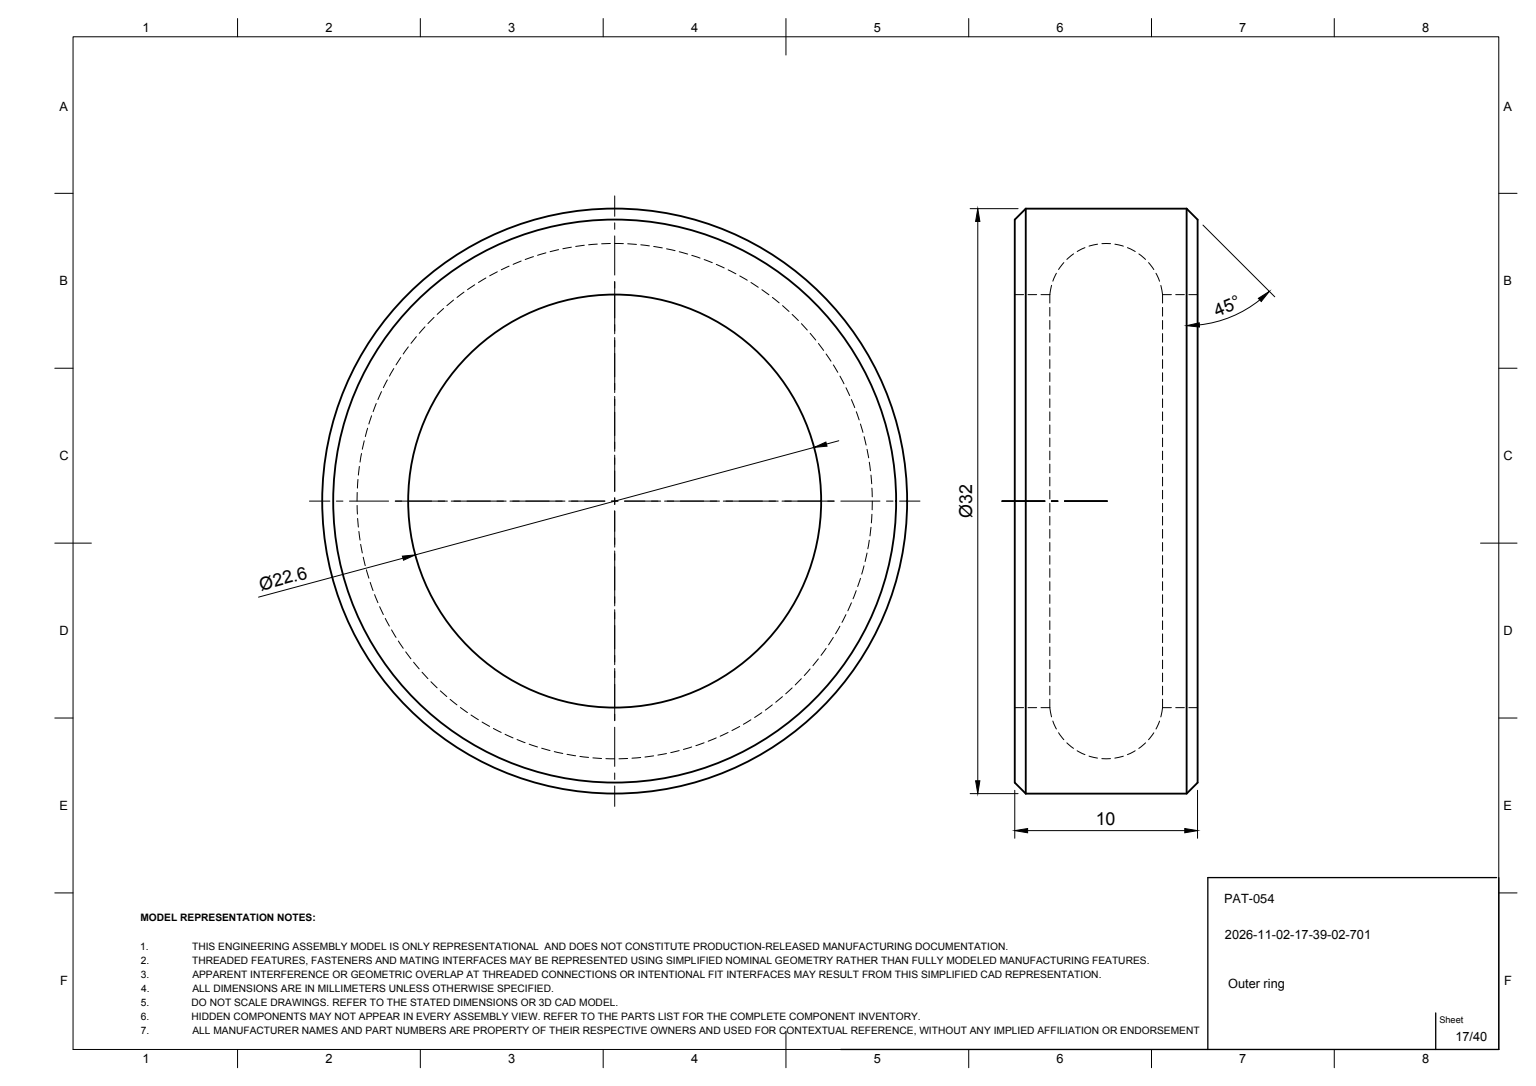
ISO-10303-21;
HEADER;
/* Generated by software containing ST-Developer
 * from STEP Tools, Inc. (www.steptools.com) 
 */

FILE_DESCRIPTION(
/* description */ ('PAT-054'),
/* implementation_level */ '2;1');

FILE_NAME(
/* name */ 'Outer ring.step',
/* time_stamp */ '2026-10-29T16:38:13-07:00',
/* author */ (''),
/* organization */ (''),
/* preprocessor_version */ 'ST-DEVELOPER v20.2',
/* originating_system */ 'Autodesk Translation Framework v15.17.0.0',
/* authorisation */ '');

FILE_SCHEMA (('AUTOMOTIVE_DESIGN { 1 0 10303 214 3 1 1 }'));
ENDSEC;

DATA;
#10=MECHANICAL_DESIGN_GEOMETRIC_PRESENTATION_REPRESENTATION('',(#909),#33981);
#779=CONICAL_SURFACE('',#13904,1.57,0.785398163397449);
#780=CONICAL_SURFACE('',#13908,1.57,0.785398163397449);
#808=TOROIDAL_SURFACE('',#13893,1.1,0.309556);
#821=SHAPE_REPRESENTATION_RELATIONSHIP('SRR','None',#34195,#865);
#865=ADVANCED_BREP_SHAPE_REPRESENTATION('',(#968),#33943);
#909=STYLED_ITEM('',(#34517),#968);
#968=MANIFOLD_SOLID_BREP('Body1',#13020);
#1130=FACE_BOUND('',#2580,.T.);
#1131=FACE_BOUND('',#2585,.T.);
#1313=PLANE('',#13901);
#1314=PLANE('',#13910);
#1736=FACE_OUTER_BOUND('',#2577,.T.);
#1737=FACE_OUTER_BOUND('',#2578,.T.);
#1738=FACE_OUTER_BOUND('',#2579,.T.);
#1739=FACE_OUTER_BOUND('',#2581,.T.);
#1740=FACE_OUTER_BOUND('',#2582,.T.);
#1741=FACE_OUTER_BOUND('',#2583,.T.);
#1742=FACE_OUTER_BOUND('',#2584,.T.);
#1743=FACE_OUTER_BOUND('',#2586,.T.);
#2577=EDGE_LOOP('',(#9259,#9260,#9261,#9262,#9263,#9264));
#2578=EDGE_LOOP('',(#9265,#9266,#9267,#9268,#9269));
#2579=EDGE_LOOP('',(#9270));
#2580=EDGE_LOOP('',(#9271));
#2581=EDGE_LOOP('',(#9272,#9273,#9274,#9275));
#2582=EDGE_LOOP('',(#9276,#9277,#9278,#9279));
#2583=EDGE_LOOP('',(#9280,#9281,#9282,#9283));
#2584=EDGE_LOOP('',(#9284));
#2585=EDGE_LOOP('',(#9285));
#2586=EDGE_LOOP('',(#9286,#9287,#9288,#9289,#9290));
#3463=LINE('',#19315,#4397);
#3464=LINE('',#19324,#4398);
#3465=LINE('',#19328,#4399);
#3466=LINE('',#19332,#4400);
#3467=LINE('',#19335,#4401);
#4397=VECTOR('',#15800,1.129765);
#4398=VECTOR('',#15811,1.57);
#4399=VECTOR('',#15816,1.6);
#4400=VECTOR('',#15821,1.57);
#4401=VECTOR('',#15826,1.129765);
#5264=CIRCLE('',#13894,1.129765);
#5265=CIRCLE('',#13895,1.129765);
#5266=CIRCLE('',#13896,0.309556);
#5267=CIRCLE('',#13897,1.129765);
#5268=CIRCLE('',#13898,1.129765);
#5269=CIRCLE('',#13900,1.129765);
#5270=CIRCLE('',#13902,1.54);
#5271=CIRCLE('',#13903,1.129765);
#5272=CIRCLE('',#13905,1.6);
#5273=CIRCLE('',#13907,1.6);
#5274=CIRCLE('',#13909,1.54);
#5826=VERTEX_POINT('',#19303);
#5827=VERTEX_POINT('',#19304);
#5828=VERTEX_POINT('',#19307);
#5829=VERTEX_POINT('',#19309);
#5830=VERTEX_POINT('',#19313);
#5831=VERTEX_POINT('',#19317);
#5832=VERTEX_POINT('',#19319);
#5833=VERTEX_POINT('',#19322);
#5834=VERTEX_POINT('',#19326);
#5835=VERTEX_POINT('',#19330);
#7129=EDGE_CURVE('',#5826,#5827,#5264,.T.);
#7130=EDGE_CURVE('',#5827,#5826,#5265,.T.);
#7131=EDGE_CURVE('',#5827,#5828,#5266,.T.);
#7132=EDGE_CURVE('',#5829,#5828,#5267,.T.);
#7133=EDGE_CURVE('',#5828,#5829,#5268,.T.);
#7134=EDGE_CURVE('',#5830,#5830,#5269,.T.);
#7135=EDGE_CURVE('',#5830,#5829,#3463,.T.);
#7136=EDGE_CURVE('',#5831,#5831,#5270,.T.);
#7137=EDGE_CURVE('',#5832,#5832,#5271,.T.);
#7138=EDGE_CURVE('',#5833,#5833,#5272,.T.);
#7139=EDGE_CURVE('',#5833,#5831,#3464,.T.);
#7140=EDGE_CURVE('',#5834,#5834,#5273,.T.);
#7141=EDGE_CURVE('',#5834,#5833,#3465,.T.);
#7142=EDGE_CURVE('',#5835,#5835,#5274,.T.);
#7143=EDGE_CURVE('',#5835,#5834,#3466,.T.);
#7144=EDGE_CURVE('',#5826,#5832,#3467,.T.);
#9259=ORIENTED_EDGE('',*,*,#7129,.F.);
#9260=ORIENTED_EDGE('',*,*,#7130,.F.);
#9261=ORIENTED_EDGE('',*,*,#7131,.T.);
#9262=ORIENTED_EDGE('',*,*,#7132,.F.);
#9263=ORIENTED_EDGE('',*,*,#7133,.F.);
#9264=ORIENTED_EDGE('',*,*,#7131,.F.);
#9265=ORIENTED_EDGE('',*,*,#7134,.T.);
#9266=ORIENTED_EDGE('',*,*,#7135,.T.);
#9267=ORIENTED_EDGE('',*,*,#7132,.T.);
#9268=ORIENTED_EDGE('',*,*,#7133,.T.);
#9269=ORIENTED_EDGE('',*,*,#7135,.F.);
#9270=ORIENTED_EDGE('',*,*,#7136,.F.);
#9271=ORIENTED_EDGE('',*,*,#7137,.T.);
#9272=ORIENTED_EDGE('',*,*,#7138,.F.);
#9273=ORIENTED_EDGE('',*,*,#7139,.T.);
#9274=ORIENTED_EDGE('',*,*,#7136,.T.);
#9275=ORIENTED_EDGE('',*,*,#7139,.F.);
#9276=ORIENTED_EDGE('',*,*,#7140,.F.);
#9277=ORIENTED_EDGE('',*,*,#7141,.T.);
#9278=ORIENTED_EDGE('',*,*,#7138,.T.);
#9279=ORIENTED_EDGE('',*,*,#7141,.F.);
#9280=ORIENTED_EDGE('',*,*,#7142,.F.);
#9281=ORIENTED_EDGE('',*,*,#7143,.T.);
#9282=ORIENTED_EDGE('',*,*,#7140,.T.);
#9283=ORIENTED_EDGE('',*,*,#7143,.F.);
#9284=ORIENTED_EDGE('',*,*,#7142,.T.);
#9285=ORIENTED_EDGE('',*,*,#7134,.F.);
#9286=ORIENTED_EDGE('',*,*,#7129,.T.);
#9287=ORIENTED_EDGE('',*,*,#7130,.T.);
#9288=ORIENTED_EDGE('',*,*,#7144,.T.);
#9289=ORIENTED_EDGE('',*,*,#7137,.F.);
#9290=ORIENTED_EDGE('',*,*,#7144,.F.);
#12052=CYLINDRICAL_SURFACE('',#13899,1.129765);
#12053=CYLINDRICAL_SURFACE('',#13906,1.6);
#12054=CYLINDRICAL_SURFACE('',#13911,1.129765);
#12448=ADVANCED_FACE('',(#1736),#808,.F.);
#12449=ADVANCED_FACE('',(#1737),#12052,.F.);
#12450=ADVANCED_FACE('',(#1738,#1130),#1313,.T.);
#12451=ADVANCED_FACE('',(#1739),#779,.T.);
#12452=ADVANCED_FACE('',(#1740),#12053,.T.);
#12453=ADVANCED_FACE('',(#1741),#780,.T.);
#12454=ADVANCED_FACE('',(#1742,#1131),#1314,.T.);
#12455=ADVANCED_FACE('',(#1743),#12054,.F.);
#13020=CLOSED_SHELL('',(#12448,#12449,#12450,#12451,#12452,#12453,#12454,
#12455));
#13892=AXIS2_PLACEMENT_3D('',#19301,#15782,#15783);
#13893=AXIS2_PLACEMENT_3D('',#19302,#15784,#15785);
#13894=AXIS2_PLACEMENT_3D('',#19305,#15786,#15787);
#13895=AXIS2_PLACEMENT_3D('',#19306,#15788,#15789);
#13896=AXIS2_PLACEMENT_3D('',#19308,#15790,#15791);
#13897=AXIS2_PLACEMENT_3D('',#19310,#15792,#15793);
#13898=AXIS2_PLACEMENT_3D('',#19311,#15794,#15795);
#13899=AXIS2_PLACEMENT_3D('',#19312,#15796,#15797);
#13900=AXIS2_PLACEMENT_3D('',#19314,#15798,#15799);
#13901=AXIS2_PLACEMENT_3D('',#19316,#15801,#15802);
#13902=AXIS2_PLACEMENT_3D('',#19318,#15803,#15804);
#13903=AXIS2_PLACEMENT_3D('',#19320,#15805,#15806);
#13904=AXIS2_PLACEMENT_3D('',#19321,#15807,#15808);
#13905=AXIS2_PLACEMENT_3D('',#19323,#15809,#15810);
#13906=AXIS2_PLACEMENT_3D('',#19325,#15812,#15813);
#13907=AXIS2_PLACEMENT_3D('',#19327,#15814,#15815);
#13908=AXIS2_PLACEMENT_3D('',#19329,#15817,#15818);
#13909=AXIS2_PLACEMENT_3D('',#19331,#15819,#15820);
#13910=AXIS2_PLACEMENT_3D('',#19333,#15822,#15823);
#13911=AXIS2_PLACEMENT_3D('',#19334,#15824,#15825);
#15782=DIRECTION('axis',(0.,0.,1.));
#15783=DIRECTION('refdir',(1.,0.,0.));
#15784=DIRECTION('center_axis',(0.,-1.,0.));
#15785=DIRECTION('ref_axis',(0.,0.,-1.));
#15786=DIRECTION('center_axis',(0.,-1.,0.));
#15787=DIRECTION('ref_axis',(1.,0.,0.));
#15788=DIRECTION('center_axis',(0.,-1.,0.));
#15789=DIRECTION('ref_axis',(1.,0.,0.));
#15790=DIRECTION('center_axis',(1.,0.,1.22464679914735E-16));
#15791=DIRECTION('ref_axis',(-1.22464679914735E-16,0.,1.));
#15792=DIRECTION('center_axis',(0.,1.,0.));
#15793=DIRECTION('ref_axis',(1.,0.,0.));
#15794=DIRECTION('center_axis',(0.,1.,0.));
#15795=DIRECTION('ref_axis',(1.,0.,0.));
#15796=DIRECTION('center_axis',(0.,-1.,0.));
#15797=DIRECTION('ref_axis',(1.,0.,0.));
#15798=DIRECTION('center_axis',(0.,-1.,0.));
#15799=DIRECTION('ref_axis',(1.,0.,0.));
#15800=DIRECTION('',(0.,1.,0.));
#15801=DIRECTION('center_axis',(0.,1.,0.));
#15802=DIRECTION('ref_axis',(0.,0.,1.));
#15803=DIRECTION('center_axis',(0.,-1.,0.));
#15804=DIRECTION('ref_axis',(1.,0.,0.));
#15805=DIRECTION('center_axis',(0.,-1.,0.));
#15806=DIRECTION('ref_axis',(1.,0.,0.));
#15807=DIRECTION('center_axis',(0.,-1.,0.));
#15808=DIRECTION('ref_axis',(1.,0.,0.));
#15809=DIRECTION('center_axis',(0.,-1.,0.));
#15810=DIRECTION('ref_axis',(1.,0.,0.));
#15811=DIRECTION('',(0.707106781186548,0.707106781186547,8.65956056235494E-17));
#15812=DIRECTION('center_axis',(0.,-1.,0.));
#15813=DIRECTION('ref_axis',(1.,0.,0.));
#15814=DIRECTION('center_axis',(0.,-1.,0.));
#15815=DIRECTION('ref_axis',(1.,0.,0.));
#15816=DIRECTION('',(0.,1.,0.));
#15817=DIRECTION('center_axis',(0.,1.,0.));
#15818=DIRECTION('ref_axis',(1.,0.,0.));
#15819=DIRECTION('center_axis',(0.,-1.,0.));
#15820=DIRECTION('ref_axis',(1.,0.,0.));
#15821=DIRECTION('',(-0.707106781186548,0.707106781186547,-8.65956056235494E-17));
#15822=DIRECTION('center_axis',(0.,-1.,0.));
#15823=DIRECTION('ref_axis',(0.,0.,-1.));
#15824=DIRECTION('center_axis',(0.,-1.,0.));
#15825=DIRECTION('ref_axis',(1.,0.,0.));
#15826=DIRECTION('',(0.,1.,0.));
#19301=CARTESIAN_POINT('',(0.,0.,0.));
#19302=CARTESIAN_POINT('Origin',(0.,0.,0.));
#19303=CARTESIAN_POINT('',(-1.129765,0.308121667383195,-1.38356309103871E-16));
#19304=CARTESIAN_POINT('',(-1.38356309103871E-16,0.308121667383195,1.129765));
#19305=CARTESIAN_POINT('Origin',(0.,0.308121667383195,0.));
#19306=CARTESIAN_POINT('Origin',(0.,0.308121667383195,0.));
#19307=CARTESIAN_POINT('',(-1.38356309103871E-16,-0.308121667383195,1.129765));
#19308=CARTESIAN_POINT('Origin',(-1.34711147906209E-16,0.,1.1));
#19309=CARTESIAN_POINT('',(-1.129765,-0.308121667383195,1.38356309103871E-16));
#19310=CARTESIAN_POINT('Origin',(0.,-0.308121667383195,0.));
#19311=CARTESIAN_POINT('Origin',(0.,-0.308121667383195,0.));
#19312=CARTESIAN_POINT('Origin',(0.,0.,0.));
#19313=CARTESIAN_POINT('',(-1.129765,-0.5,-1.38356309103871E-16));
#19314=CARTESIAN_POINT('Origin',(0.,-0.5,0.));
#19315=CARTESIAN_POINT('',(-1.129765,0.,-1.38356309103871E-16));
#19316=CARTESIAN_POINT('Origin',(1.54,0.5,0.));
#19317=CARTESIAN_POINT('',(-1.54,0.5,-1.88595607068692E-16));
#19318=CARTESIAN_POINT('Origin',(0.,0.5,0.));
#19319=CARTESIAN_POINT('',(-1.129765,0.5,-1.38356309103871E-16));
#19320=CARTESIAN_POINT('Origin',(0.,0.5,0.));
#19321=CARTESIAN_POINT('Origin',(0.,0.47,0.));
#19322=CARTESIAN_POINT('',(-1.6,0.44,-1.95943487863577E-16));
#19323=CARTESIAN_POINT('Origin',(0.,0.44,0.));
#19324=CARTESIAN_POINT('',(-1.57,0.47,-1.92269547466134E-16));
#19325=CARTESIAN_POINT('Origin',(0.,0.,0.));
#19326=CARTESIAN_POINT('',(-1.6,-0.44,-1.95943487863577E-16));
#19327=CARTESIAN_POINT('Origin',(0.,-0.44,0.));
#19328=CARTESIAN_POINT('',(-1.6,0.,-1.95943487863577E-16));
#19329=CARTESIAN_POINT('Origin',(0.,-0.47,0.));
#19330=CARTESIAN_POINT('',(-1.54,-0.5,-1.88595607068692E-16));
#19331=CARTESIAN_POINT('Origin',(0.,-0.5,0.));
#19332=CARTESIAN_POINT('',(-1.57,-0.47,-1.92269547466134E-16));
#19333=CARTESIAN_POINT('Origin',(1.129765,-0.5,0.));
#19334=CARTESIAN_POINT('Origin',(0.,0.,0.));
#19335=CARTESIAN_POINT('',(-1.129765,0.,-1.38356309103871E-16));
#33891=UNCERTAINTY_MEASURE_WITH_UNIT(LENGTH_MEASURE(0.001),#33982,
'DISTANCE_ACCURACY_VALUE',
'Maximum model space distance between geometric entities at asserted c
onnectivities');
#33929=UNCERTAINTY_MEASURE_WITH_UNIT(LENGTH_MEASURE(0.001),#33982,
'DISTANCE_ACCURACY_VALUE',
'Maximum model space distance between geometric entities at asserted c
onnectivities');
#33943=(
GEOMETRIC_REPRESENTATION_CONTEXT(3)
GLOBAL_UNCERTAINTY_ASSIGNED_CONTEXT((#33891))
GLOBAL_UNIT_ASSIGNED_CONTEXT((#33982,#33984,#33985))
REPRESENTATION_CONTEXT('','3D')
);
#33981=(
GEOMETRIC_REPRESENTATION_CONTEXT(3)
GLOBAL_UNCERTAINTY_ASSIGNED_CONTEXT((#33929))
GLOBAL_UNIT_ASSIGNED_CONTEXT((#33982,#33984,#33985))
REPRESENTATION_CONTEXT('','3D')
);
#33982=(
LENGTH_UNIT()
NAMED_UNIT(*)
SI_UNIT(.CENTI.,.METRE.)
);
#33984=(
NAMED_UNIT(*)
PLANE_ANGLE_UNIT()
SI_UNIT($,.RADIAN.)
);
#33985=(
NAMED_UNIT(*)
SI_UNIT($,.STERADIAN.)
SOLID_ANGLE_UNIT()
);
#33999=SHAPE_DEFINITION_REPRESENTATION(#34050,#34195);
#34050=PRODUCT_DEFINITION_SHAPE('',$,#34247);
#34195=SHAPE_REPRESENTATION('',(#13892),#33943);
#34233=PRODUCT_DEFINITION_CONTEXT('part definition',#34388,'design');
#34247=PRODUCT_DEFINITION('Outer ring','Outer ring',#34298,#34233);
#34298=PRODUCT_DEFINITION_FORMATION('',$,#34403);
#34388=APPLICATION_CONTEXT(
'Core Data for Automotive Mechanical Design Process');
#34389=PRODUCT_CONTEXT('part definition',#34388,'mechanical');
#34403=PRODUCT('Outer ring','Outer ring','Outer ring',(#34389));
#34511=COLOUR_RGB('Grey',0.48,0.52,0.57);
#34512=FILL_AREA_STYLE_COLOUR('',#34511);
#34513=FILL_AREA_STYLE('',(#34512));
#34514=SURFACE_STYLE_FILL_AREA(#34513);
#34515=SURFACE_SIDE_STYLE('',(#34514));
#34516=SURFACE_STYLE_USAGE(.BOTH.,#34515);
#34517=PRESENTATION_STYLE_ASSIGNMENT((#34516));
ENDSEC;
END-ISO-10303-21;
